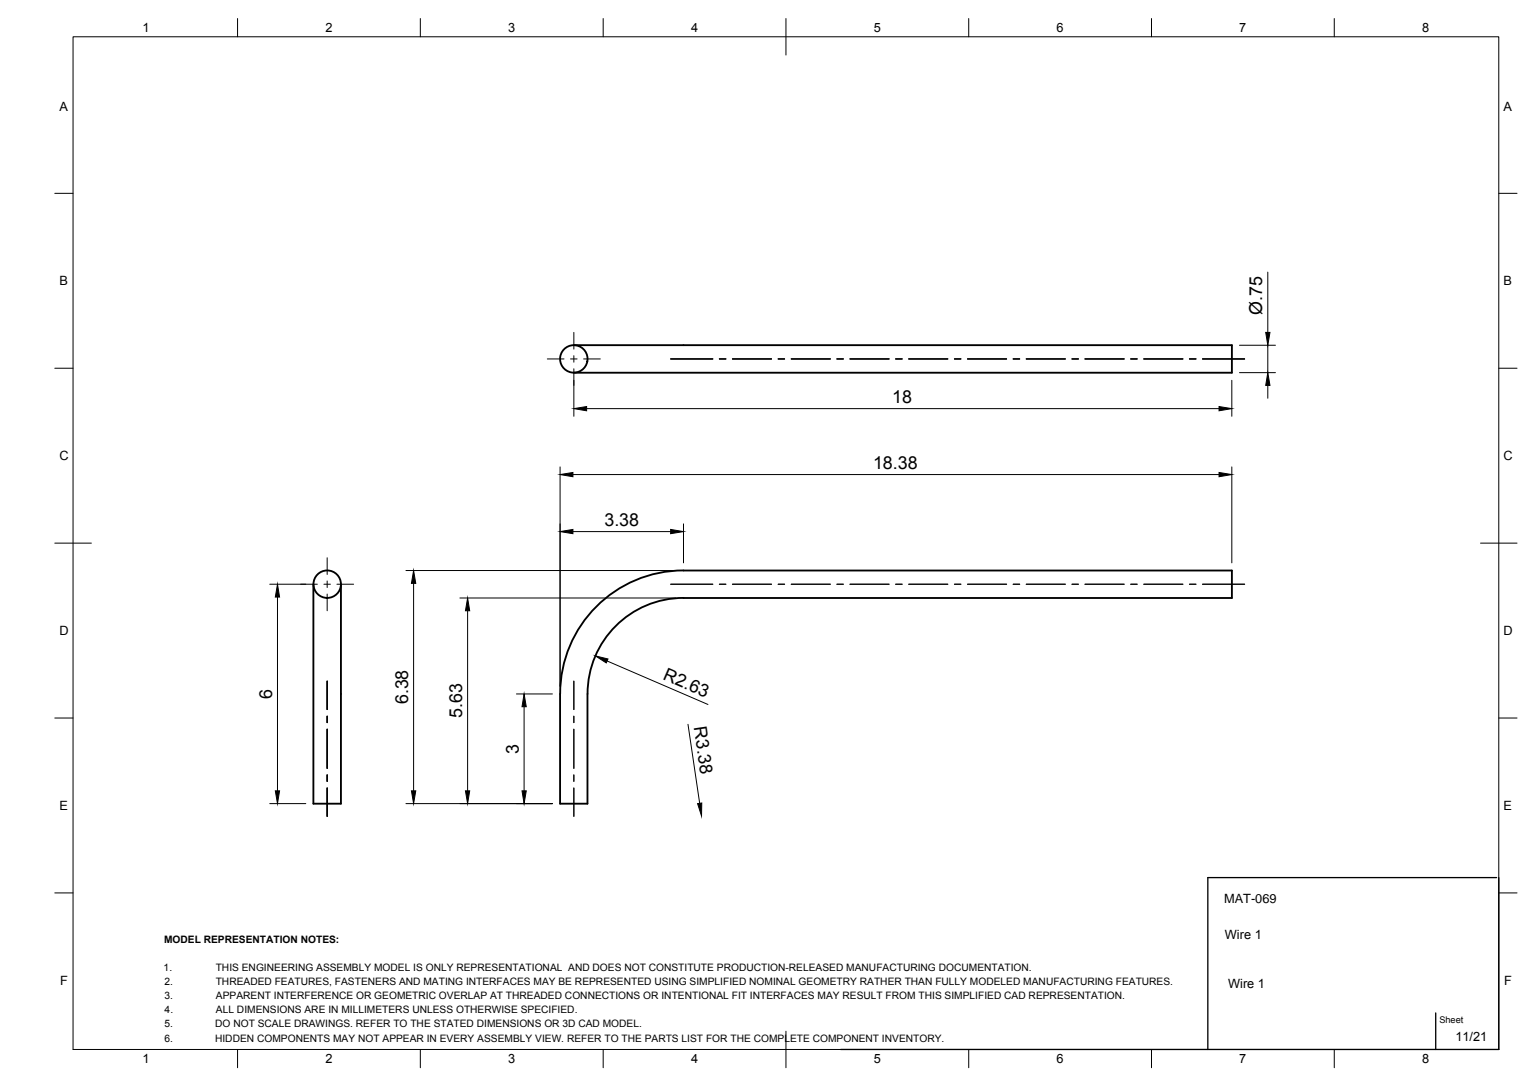
ISO-10303-21;
HEADER;
/* Generated by software containing ST-Developer
 * from STEP Tools, Inc. (www.steptools.com) 
 */

FILE_DESCRIPTION(
/* description */ ('CAx-IF Rec.Pracs.---Representation and Presentation of Product Manufa
cturing Information (PMI)---4.0---2014-10-13'),
/* implementation_level */ '2;1');

FILE_NAME(
/* name */ 'Wire 1.step',
/* time_stamp */ '2026-10-24T15:08:39-07:00',
/* author */ (''),
/* organization */ (''),
/* preprocessor_version */ 'ST-DEVELOPER v20.2',
/* originating_system */ 'Autodesk Translation Framework v15.17.0.0',
/* authorisation */ '');

FILE_SCHEMA (('AP242_MANAGED_MODEL_BASED_3D_ENGINEERING_MIM_LF { 1 0 10303 442 2 1 4 }'));
ENDSEC;

DATA;
#10=MECHANICAL_DESIGN_GEOMETRIC_PRESENTATION_REPRESENTATION('',(#828),#50081);
#775=TOROIDAL_SURFACE('',#10458,0.003,0.000375);
#788=SHAPE_REPRESENTATION_RELATIONSHIP('SRR','None',#50156,#808);
#808=ADVANCED_BREP_SHAPE_REPRESENTATION('',(#848),#50069);
#828=STYLED_ITEM('',(#50260),#848);
#848=MANIFOLD_SOLID_BREP('Body1',#9873);
#958=PLANE('',#10464);
#959=PLANE('',#10465);
#1271=FACE_OUTER_BOUND('',#1843,.T.);
#1272=FACE_OUTER_BOUND('',#1844,.T.);
#1273=FACE_OUTER_BOUND('',#1845,.T.);
#1274=FACE_OUTER_BOUND('',#1846,.T.);
#1275=FACE_OUTER_BOUND('',#1847,.T.);
#1843=EDGE_LOOP('',(#7034,#7035,#7036,#7037,#7038));
#1844=EDGE_LOOP('',(#7039,#7040,#7041,#7042,#7043,#7044));
#1845=EDGE_LOOP('',(#7045,#7046,#7047,#7048,#7049));
#1846=EDGE_LOOP('',(#7050));
#1847=EDGE_LOOP('',(#7051));
#2401=LINE('',#18123,#2979);
#2402=LINE('',#18135,#2980);
#2979=VECTOR('',#11893,0.000375);
#2980=VECTOR('',#11908,0.000375);
#3552=CIRCLE('',#10455,0.00037500000001);
#3553=CIRCLE('',#10456,0.00037500000001);
#3554=CIRCLE('',#10457,0.00037500000001);
#3555=CIRCLE('',#10459,0.002625);
#3556=CIRCLE('',#10460,0.00037500000001);
#3557=CIRCLE('',#10461,0.00037500000001);
#3558=CIRCLE('',#10463,0.00037500000001);
#4050=VERTEX_POINT('',#18120);
#4051=VERTEX_POINT('',#18122);
#4052=VERTEX_POINT('',#18124);
#4053=VERTEX_POINT('',#18128);
#4054=VERTEX_POINT('',#18130);
#4055=VERTEX_POINT('',#18134);
#5170=EDGE_CURVE('',#4050,#4050,#3552,.T.);
#5171=EDGE_CURVE('',#4050,#4051,#2401,.T.);
#5172=EDGE_CURVE('',#4051,#4052,#3553,.T.);
#5173=EDGE_CURVE('',#4052,#4051,#3554,.T.);
#5174=EDGE_CURVE('',#4052,#4053,#3555,.T.);
#5175=EDGE_CURVE('',#4053,#4054,#3556,.T.);
#5176=EDGE_CURVE('',#4054,#4053,#3557,.T.);
#5177=EDGE_CURVE('',#4054,#4055,#2402,.T.);
#5178=EDGE_CURVE('',#4055,#4055,#3558,.T.);
#7034=ORIENTED_EDGE('',*,*,#5170,.F.);
#7035=ORIENTED_EDGE('',*,*,#5171,.T.);
#7036=ORIENTED_EDGE('',*,*,#5172,.T.);
#7037=ORIENTED_EDGE('',*,*,#5173,.T.);
#7038=ORIENTED_EDGE('',*,*,#5171,.F.);
#7039=ORIENTED_EDGE('',*,*,#5173,.F.);
#7040=ORIENTED_EDGE('',*,*,#5174,.T.);
#7041=ORIENTED_EDGE('',*,*,#5175,.T.);
#7042=ORIENTED_EDGE('',*,*,#5176,.T.);
#7043=ORIENTED_EDGE('',*,*,#5174,.F.);
#7044=ORIENTED_EDGE('',*,*,#5172,.F.);
#7045=ORIENTED_EDGE('',*,*,#5176,.F.);
#7046=ORIENTED_EDGE('',*,*,#5177,.T.);
#7047=ORIENTED_EDGE('',*,*,#5178,.T.);
#7048=ORIENTED_EDGE('',*,*,#5177,.F.);
#7049=ORIENTED_EDGE('',*,*,#5175,.F.);
#7050=ORIENTED_EDGE('',*,*,#5170,.T.);
#7051=ORIENTED_EDGE('',*,*,#5178,.F.);
#9184=CYLINDRICAL_SURFACE('',#10454,0.000375);
#9185=CYLINDRICAL_SURFACE('',#10462,0.000375);
#9493=ADVANCED_FACE('',(#1271),#9184,.T.);
#9494=ADVANCED_FACE('',(#1272),#775,.T.);
#9495=ADVANCED_FACE('',(#1273),#9185,.T.);
#9496=ADVANCED_FACE('',(#1274),#958,.T.);
#9497=ADVANCED_FACE('',(#1275),#959,.F.);
#9873=CLOSED_SHELL('',(#9493,#9494,#9495,#9496,#9497));
#10453=AXIS2_PLACEMENT_3D('',#18118,#11887,#11888);
#10454=AXIS2_PLACEMENT_3D('',#18119,#11889,#11890);
#10455=AXIS2_PLACEMENT_3D('',#18121,#11891,#11892);
#10456=AXIS2_PLACEMENT_3D('',#18125,#11894,#11895);
#10457=AXIS2_PLACEMENT_3D('',#18126,#11896,#11897);
#10458=AXIS2_PLACEMENT_3D('',#18127,#11898,#11899);
#10459=AXIS2_PLACEMENT_3D('',#18129,#11900,#11901);
#10460=AXIS2_PLACEMENT_3D('',#18131,#11902,#11903);
#10461=AXIS2_PLACEMENT_3D('',#18132,#11904,#11905);
#10462=AXIS2_PLACEMENT_3D('',#18133,#11906,#11907);
#10463=AXIS2_PLACEMENT_3D('',#18136,#11909,#11910);
#10464=AXIS2_PLACEMENT_3D('',#18137,#11911,#11912);
#10465=AXIS2_PLACEMENT_3D('',#18138,#11913,#11914);
#11887=DIRECTION('axis',(0.,0.,1.));
#11888=DIRECTION('refdir',(1.,0.,0.));
#11889=DIRECTION('center_axis',(-6.74488507274914E-15,1.49880108324396E-15,
-1.));
#11890=DIRECTION('ref_axis',(-0.173648177666927,-0.984807753012209,-3.04793925546002E-16));
#11891=DIRECTION('center_axis',(2.62550741678841E-11,-4.62916846043658E-12,
-1.));
#11892=DIRECTION('ref_axis',(-0.173648177666927,-0.984807753012209,-3.04793925548737E-16));
#11893=DIRECTION('',(6.74488507274914E-15,-1.49880108324396E-15,1.));
#11894=DIRECTION('center_axis',(2.62550741678841E-11,-4.62916846043658E-12,
-1.));
#11895=DIRECTION('ref_axis',(-0.173648177666927,-0.984807753012209,-3.04793925548737E-16));
#11896=DIRECTION('center_axis',(2.62550741678841E-11,-4.62916846043658E-12,
-1.));
#11897=DIRECTION('ref_axis',(-0.173648177666927,-0.984807753012209,-3.04793925548737E-16));
#11898=DIRECTION('center_axis',(0.173648177666927,0.984807753012209,1.41609297436625E-15));
#11899=DIRECTION('ref_axis',(-6.16790569236198E-15,2.05596856412066E-15,
-1.));
#11900=DIRECTION('center_axis',(-0.173648177666927,-0.984807753012209,-1.41609297436625E-15));
#11901=DIRECTION('ref_axis',(-5.78605122952035E-15,2.45817543460173E-15,
-1.));
#11902=DIRECTION('center_axis',(0.984807753012209,-0.173648177666927,-6.9026791896102E-15));
#11903=DIRECTION('ref_axis',(-0.173648177666927,-0.984807753012209,-1.41609297436625E-15));
#11904=DIRECTION('center_axis',(0.984807753012209,-0.173648177666927,-6.9026791896102E-15));
#11905=DIRECTION('ref_axis',(-0.173648177666927,-0.984807753012209,-1.41609297436625E-15));
#11906=DIRECTION('center_axis',(0.984807753012209,-0.173648177666927,-6.9026791896102E-15));
#11907=DIRECTION('ref_axis',(-0.173648177666927,-0.984807753012209,-1.41609297436625E-15));
#11908=DIRECTION('',(-0.984807753012209,0.173648177666927,6.9026791896102E-15));
#11909=DIRECTION('center_axis',(0.984807753012209,-0.173648177666927,-6.9026791896102E-15));
#11910=DIRECTION('ref_axis',(-0.173648177666927,-0.984807753012209,-1.41609297436625E-15));
#11911=DIRECTION('center_axis',(-6.46591174117934E-15,1.44961055799008E-15,
-1.));
#11912=DIRECTION('ref_axis',(-0.173648177666927,-0.984807753012209,-3.04793925546006E-16));
#11913=DIRECTION('center_axis',(0.984807753012209,-0.173648177666927,-6.9026791896102E-15));
#11914=DIRECTION('ref_axis',(6.74488507274914E-15,-1.49880108324396E-15,
1.));
#18118=CARTESIAN_POINT('',(0.,0.,0.));
#18119=CARTESIAN_POINT('Origin',(-0.00623952773349959,-0.035801562760354,
0.000824146758145402));
#18120=CARTESIAN_POINT('',(-0.00617440966687451,-0.0354322598529744,-0.00217585328655807));
#18121=CARTESIAN_POINT('Origin',(-0.00623952773350945,-0.0358015627603522,
-0.00217585328654807));
#18122=CARTESIAN_POINT('',(-0.00617440966687449,-0.0354322598529744,0.000824146758165403));
#18123=CARTESIAN_POINT('',(-0.00617440966687449,-0.0354322598529744,0.000824146758145402));
#18124=CARTESIAN_POINT('',(-0.00660883064089887,-0.0357364446937254,0.000824146758145405));
#18125=CARTESIAN_POINT('Origin',(-0.00623952773350944,-0.0358015627603522,
0.000824146758155403));
#18126=CARTESIAN_POINT('Origin',(-0.00623952773350944,-0.0358015627603522,
0.000824146758155403));
#18127=CARTESIAN_POINT('Origin',(-0.00919395099253621,-0.0352806182273532,
0.000824146758145423));
#18128=CARTESIAN_POINT('',(-0.00919395099254605,-0.0352806182273515,0.00344914675814542));
#18129=CARTESIAN_POINT('Origin',(-0.00919395099253621,-0.0352806182273532,
0.000824146758145423));
#18130=CARTESIAN_POINT('',(-0.00912883292592094,-0.0349113153199719,0.00382414675814543));
#18131=CARTESIAN_POINT('Origin',(-0.00919395099254604,-0.0352806182273514,
0.00382414675815542));
#18132=CARTESIAN_POINT('Origin',(-0.00919395099254604,-0.0352806182273514,
0.00382414675815542));
#18133=CARTESIAN_POINT('Origin',(-0.0239660672877193,-0.0326758955623493,
0.00382414675814553));
#18134=CARTESIAN_POINT('',(-0.0239009492211041,-0.032306592654968,0.00382414675814553));
#18135=CARTESIAN_POINT('',(-0.0239009492210942,-0.0323065926549697,0.00382414675814553));
#18136=CARTESIAN_POINT('Origin',(-0.0239660672877292,-0.0326758955623476,
0.00382414675815552));
#18137=CARTESIAN_POINT('Origin',(-0.00623952773349961,-0.035801562760354,
-0.00217585328655807));
#18138=CARTESIAN_POINT('Origin',(-0.0239660672877193,-0.0326758955623493,
0.00382414675814553));
#50047=UNCERTAINTY_MEASURE_WITH_UNIT(LENGTH_MEASURE(1.E-5),#50082,
'DISTANCE_ACCURACY_VALUE',
'Maximum model space distance between geometric entities at asserted c
onnectivities');
#50059=UNCERTAINTY_MEASURE_WITH_UNIT(LENGTH_MEASURE(1.E-5),#50082,
'DISTANCE_ACCURACY_VALUE',
'Maximum model space distance between geometric entities at asserted c
onnectivities');
#50069=(
GEOMETRIC_REPRESENTATION_CONTEXT(3)
GLOBAL_UNCERTAINTY_ASSIGNED_CONTEXT((#50047))
GLOBAL_UNIT_ASSIGNED_CONTEXT((#50082,#50083,#50084))
REPRESENTATION_CONTEXT('','3D')
);
#50081=(
GEOMETRIC_REPRESENTATION_CONTEXT(3)
GLOBAL_UNCERTAINTY_ASSIGNED_CONTEXT((#50059))
GLOBAL_UNIT_ASSIGNED_CONTEXT((#50082,#50083,#50084))
REPRESENTATION_CONTEXT('','3D')
);
#50082=(
LENGTH_UNIT()
NAMED_UNIT(*)
SI_UNIT($,.METRE.)
);
#50083=(
NAMED_UNIT(*)
PLANE_ANGLE_UNIT()
SI_UNIT($,.RADIAN.)
);
#50084=(
NAMED_UNIT(*)
SI_UNIT($,.STERADIAN.)
SOLID_ANGLE_UNIT()
);
#50094=SHAPE_DEFINITION_REPRESENTATION(#50115,#50156);
#50115=PRODUCT_DEFINITION_SHAPE('',$,#50178);
#50156=SHAPE_REPRESENTATION('',(#10453),#50069);
#50168=PRODUCT_DEFINITION_CONTEXT('part definition',#50233,'design');
#50178=PRODUCT_DEFINITION('Wire 1','Wire 1',#50199,#50168);
#50199=PRODUCT_DEFINITION_FORMATION('',$,#50244);
#50233=APPLICATION_CONTEXT('Managed model based 3d engineering');
#50234=PRODUCT_CONTEXT('part definition',#50233,'mechanical');
#50244=PRODUCT('Wire 1','Wire 1','Wire_1',(#50234));
#50260=PRESENTATION_STYLE_ASSIGNMENT((#50267));
#50267=SURFACE_STYLE_USAGE(.BOTH.,#50274);
#50274=SURFACE_SIDE_STYLE('',(#50281));
#50281=SURFACE_STYLE_FILL_AREA(#50288);
#50288=FILL_AREA_STYLE('Opaque(25,25,25)',(#50295));
#50295=FILL_AREA_STYLE_COLOUR('Opaque(25,25,25)',#50302);
#50302=COLOUR_RGB('Opaque(25,25,25)',0.0980392156862745,0.0980392156862745,
0.0980392156862745);
ENDSEC;
END-ISO-10303-21;
